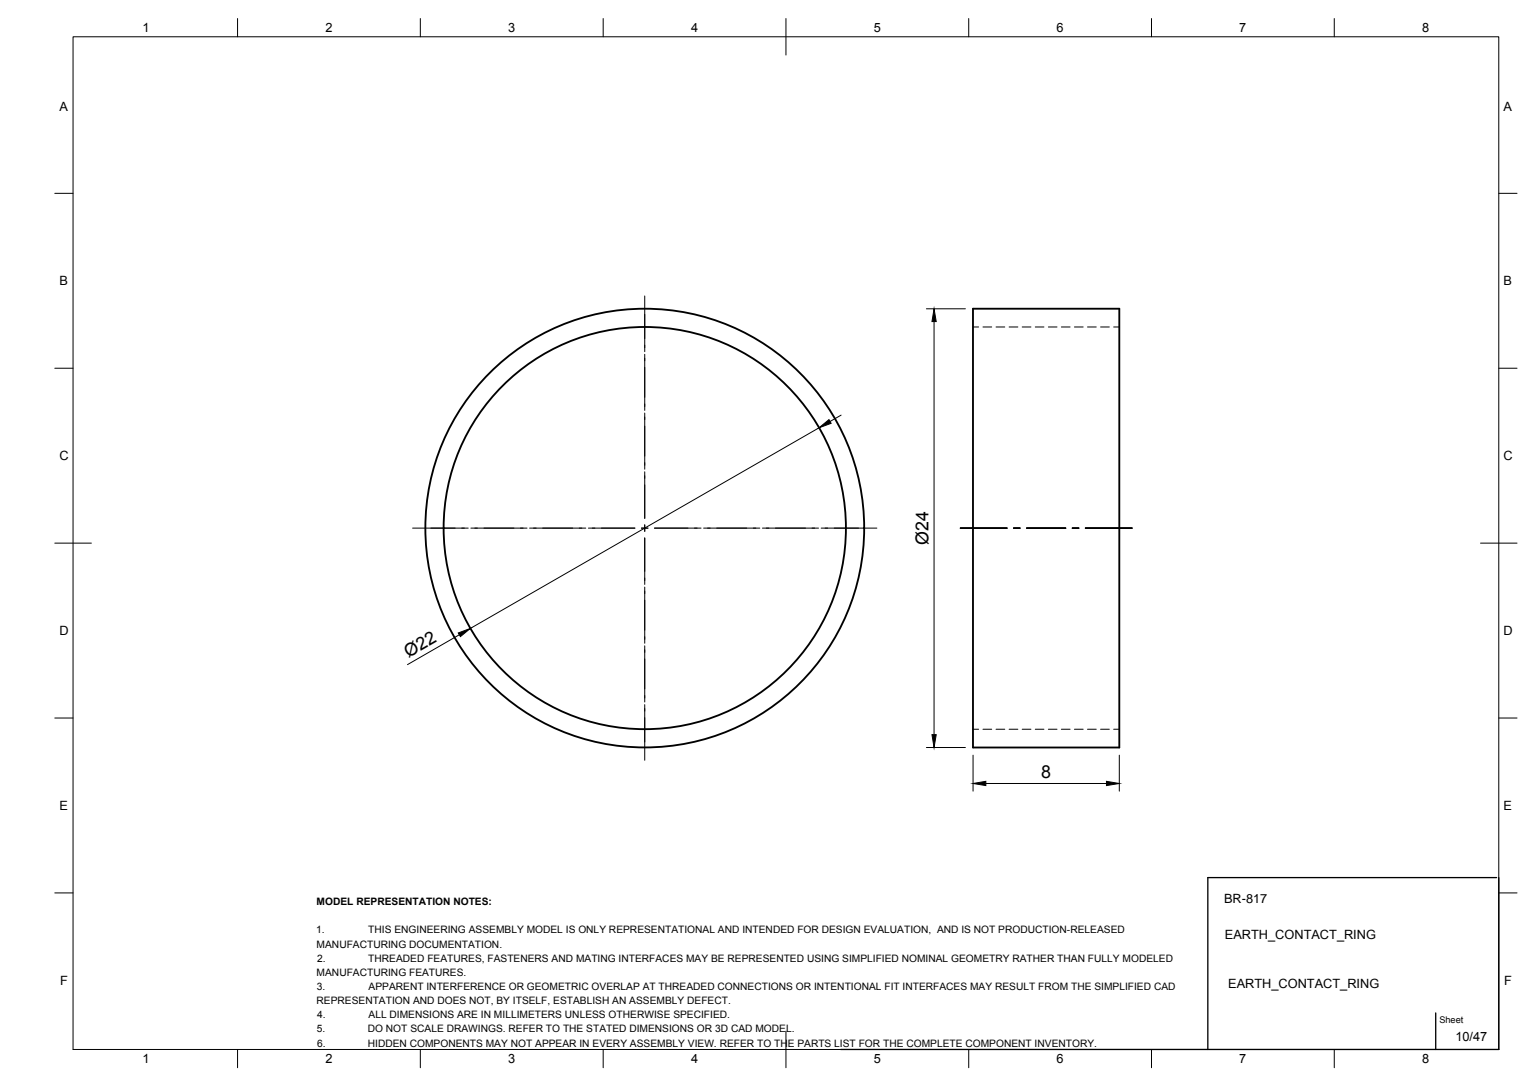
ISO-10303-21;
HEADER;
FILE_DESCRIPTION((''),'2;1');
FILE_NAME('EARTH_CONTACT_RING.step','2026-10-01T22:07:29-07:00',(''),(''),'','','');
FILE_SCHEMA (('AUTOMOTIVE_DESIGN { 1 0 10303 214 3 1 1 }'));
ENDSEC;
DATA;
#10=MECHANICAL_DESIGN_GEOMETRIC_PRESENTATION_REPRESENTATION('',(#546),#15484);
#476=SHAPE_REPRESENTATION_RELATIONSHIP('SRR','None',#15624,#511) ;
#511=ADVANCED_BREP_SHAPE_REPRESENTATION('',(#588),#15448) ;
#546=STYLED_ITEM('',(#15834),#588) ;
#588=MANIFOLD_SOLID_BREP('EARTH_CONTACT_RING',#8255) ;
#652=CYLINDRICAL_SURFACE('',#8841,1.1) ;
#653=CYLINDRICAL_SURFACE('',#8844,1.2) ;
#845=FACE_BOUND('',#2001,.T.) ;
#846=FACE_BOUND('',#2003,.T.) ;
#937=CIRCLE('',#8842,1.1) ;
#938=CIRCLE('',#8843,1.1) ;
#939=CIRCLE('',#8845,1.2) ;
#940=CIRCLE('',#8846,1.2) ;
#1463=FACE_OUTER_BOUND('',#1998,.T.) ;
#1464=FACE_OUTER_BOUND('',#1999,.T.) ;
#1465=FACE_OUTER_BOUND('',#2000,.T.) ;
#1466=FACE_OUTER_BOUND('',#2002,.T.) ;
#1998=EDGE_LOOP('',(#5711,#5712,#5713,#5714)) ;
#1999=EDGE_LOOP('',(#5715,#5716,#5717,#5718)) ;
#2000=EDGE_LOOP('',(#5719)) ;
#2001=EDGE_LOOP('',(#5720)) ;
#2002=EDGE_LOOP('',(#5721)) ;
#2003=EDGE_LOOP('',(#5722)) ;
#2607=LINE('',#13361,#3081) ;
#2608=LINE('',#13367,#3082) ;
#3081=VECTOR('',#10414,1.1) ;
#3082=VECTOR('',#10421,1.2) ;
#3534=VERTEX_POINT('',#13358) ;
#3535=VERTEX_POINT('',#13360) ;
#3536=VERTEX_POINT('',#13364) ;
#3537=VERTEX_POINT('',#13366) ;
#4360=EDGE_CURVE('',#3534,#3534,#937,.T.) ;
#4361=EDGE_CURVE('',#3534,#3535,#2607,.T.) ;
#4362=EDGE_CURVE('',#3535,#3535,#938,.T.) ;
#4363=EDGE_CURVE('',#3536,#3536,#939,.T.) ;
#4364=EDGE_CURVE('',#3536,#3537,#2608,.T.) ;
#4365=EDGE_CURVE('',#3537,#3537,#940,.T.) ;
#5711=ORIENTED_EDGE('',*,*,#4360,.F.) ;
#5712=ORIENTED_EDGE('',*,*,#4361,.T.) ;
#5713=ORIENTED_EDGE('',*,*,#4362,.F.) ;
#5714=ORIENTED_EDGE('',*,*,#4361,.F.) ;
#5715=ORIENTED_EDGE('',*,*,#4363,.F.) ;
#5716=ORIENTED_EDGE('',*,*,#4364,.T.) ;
#5717=ORIENTED_EDGE('',*,*,#4365,.F.) ;
#5718=ORIENTED_EDGE('',*,*,#4364,.F.) ;
#5719=ORIENTED_EDGE('',*,*,#4365,.T.) ;
#5720=ORIENTED_EDGE('',*,*,#4360,.T.) ;
#5721=ORIENTED_EDGE('',*,*,#4363,.T.) ;
#5722=ORIENTED_EDGE('',*,*,#4362,.T.) ;
#7609=PLANE('',#8847) ;
#7610=PLANE('',#8848) ;
#7850=ADVANCED_FACE('',(#1463),#652,.F.) ;
#7851=ADVANCED_FACE('',(#1464),#653,.T.) ;
#7852=ADVANCED_FACE('',(#1465,#845),#7609,.T.) ;
#7853=ADVANCED_FACE('',(#1466,#846),#7610,.T.) ;
#8255=CLOSED_SHELL('',(#7850,#7851,#7852,#7853)) ;
#8840=AXIS2_PLACEMENT_3D('',#13356,#10408,#10409) ;
#8841=AXIS2_PLACEMENT_3D('',#13357,#10410,#10411) ;
#8842=AXIS2_PLACEMENT_3D('',#13359,#10412,#10413) ;
#8843=AXIS2_PLACEMENT_3D('',#13362,#10415,#10416) ;
#8844=AXIS2_PLACEMENT_3D('',#13363,#10417,#10418) ;
#8845=AXIS2_PLACEMENT_3D('',#13365,#10419,#10420) ;
#8846=AXIS2_PLACEMENT_3D('',#13368,#10422,#10423) ;
#8847=AXIS2_PLACEMENT_3D('',#13369,#10424,#10425) ;
#8848=AXIS2_PLACEMENT_3D('',#13370,#10426,#10427) ;
#10408=DIRECTION('axis',(0.,0.,1.)) ;
#10409=DIRECTION('refdir',(1.,0.,0.)) ;
#10410=DIRECTION('center_axis',(0.,0.,1.)) ;
#10411=DIRECTION('ref_axis',(1.,0.,0.)) ;
#10412=DIRECTION('center_axis',(0.,0.,1.)) ;
#10413=DIRECTION('ref_axis',(1.,0.,0.)) ;
#10414=DIRECTION('',(0.,0.,1.)) ;
#10415=DIRECTION('center_axis',(0.,0.,-1.)) ;
#10416=DIRECTION('ref_axis',(1.,0.,0.)) ;
#10417=DIRECTION('center_axis',(0.,0.,1.)) ;
#10418=DIRECTION('ref_axis',(1.,0.,0.)) ;
#10419=DIRECTION('center_axis',(0.,0.,1.)) ;
#10420=DIRECTION('ref_axis',(1.,0.,0.)) ;
#10421=DIRECTION('',(0.,0.,-1.)) ;
#10422=DIRECTION('center_axis',(0.,0.,-1.)) ;
#10423=DIRECTION('ref_axis',(1.,0.,0.)) ;
#10424=DIRECTION('center_axis',(0.,0.,-1.)) ;
#10425=DIRECTION('ref_axis',(-1.,0.,0.)) ;
#10426=DIRECTION('center_axis',(0.,0.,1.)) ;
#10427=DIRECTION('ref_axis',(1.,0.,0.)) ;
#13356=CARTESIAN_POINT('',(0.,0.,0.)) ;
#13357=CARTESIAN_POINT('Origin',(-1.,0.,-0.7)) ;
#13358=CARTESIAN_POINT('',(-2.1,-1.34711147906209E-16,-1.1)) ;
#13359=CARTESIAN_POINT('Origin',(-1.,0.,-1.1)) ;
#13360=CARTESIAN_POINT('',(-2.1,1.34711147906209E-16,-0.3)) ;
#13361=CARTESIAN_POINT('',(-2.1,-1.34711147906209E-16,-0.7)) ;
#13362=CARTESIAN_POINT('Origin',(-1.,0.,-0.3)) ;
#13363=CARTESIAN_POINT('Origin',(-1.,0.,-0.7)) ;
#13364=CARTESIAN_POINT('',(-2.2,-1.46957615897682E-16,-0.3)) ;
#13365=CARTESIAN_POINT('Origin',(-1.,0.,-0.3)) ;
#13366=CARTESIAN_POINT('',(-2.2,-1.46957615897682E-16,-1.1)) ;
#13367=CARTESIAN_POINT('',(-2.2,-1.46957615897682E-16,-0.7)) ;
#13368=CARTESIAN_POINT('Origin',(-1.,0.,-1.1)) ;
#13369=CARTESIAN_POINT('Origin',(-1.,0.,-1.1)) ;
#13370=CARTESIAN_POINT('Origin',(-1.,0.,-0.3)) ;
#15405=UNCERTAINTY_MEASURE_WITH_UNIT(LENGTH_MEASURE(0.001),#15485,
'DISTANCE_ACCURACY_VALUE',
'Maximum model space distance between geometric entities at asserted c
onnectivities') ;
#15441=UNCERTAINTY_MEASURE_WITH_UNIT(LENGTH_MEASURE(0.001),#15485,
'DISTANCE_ACCURACY_VALUE',
'Maximum model space distance between geometric entities at asserted c
onnectivities') ;
#15448=(
GEOMETRIC_REPRESENTATION_CONTEXT(3)
GLOBAL_UNCERTAINTY_ASSIGNED_CONTEXT((#15405))
GLOBAL_UNIT_ASSIGNED_CONTEXT((#15485,#15487,#15488))
REPRESENTATION_CONTEXT('','3D')
) ;
#15484=(
GEOMETRIC_REPRESENTATION_CONTEXT(3)
GLOBAL_UNCERTAINTY_ASSIGNED_CONTEXT((#15441))
GLOBAL_UNIT_ASSIGNED_CONTEXT((#15485,#15487,#15488))
REPRESENTATION_CONTEXT('','3D')
) ;
#15485=(
LENGTH_UNIT()
NAMED_UNIT(*)
SI_UNIT(.CENTI.,.METRE.)
) ;
#15487=(
NAMED_UNIT(*)
PLANE_ANGLE_UNIT()
SI_UNIT($,.RADIAN.)
) ;
#15488=(
NAMED_UNIT(*)
SI_UNIT($,.STERADIAN.)
SOLID_ANGLE_UNIT()
) ;
#15495=SHAPE_DEFINITION_REPRESENTATION(#15539,#15624) ;
#15539=PRODUCT_DEFINITION_SHAPE('',$,#15667) ;
#15624=SHAPE_REPRESENTATION('',(#8840),#15448) ;
#15660=PRODUCT_DEFINITION_CONTEXT('part definition',#15788,'design') ;
#15667=PRODUCT_DEFINITION('EARTH_CONTACT_RING',
'EARTH_CONTACT_RING',#15709,#15660) ;
#15709=PRODUCT_DEFINITION_FORMATION('',$,#15796) ;
#15788=APPLICATION_CONTEXT(
'Core Data for Automotive Mechanical Design Process') ;
#15789=PRODUCT_CONTEXT('part definition',#15788,'mechanical') ;
#15796=PRODUCT('EARTH_CONTACT_RING','EARTH_CONTACT_RING',$,(#15789)) ;
#15834=PRESENTATION_STYLE_ASSIGNMENT((#15846)) ;
#15846=SURFACE_STYLE_USAGE(.BOTH.,#15858) ;
#15858=SURFACE_SIDE_STYLE('',(#15870)) ;
#15870=SURFACE_STYLE_FILL_AREA(#15882) ;
#15882=FILL_AREA_STYLE('Brass - Polished',(#15894)) ;
#15894=FILL_AREA_STYLE_COLOUR('Brass - Polished',#15906) ;
#15906=COLOUR_RGB('Brass - Polished', 0.08235294, 0.09019608, 0.10196078) ;
ENDSEC;
END-ISO-10303-21;
